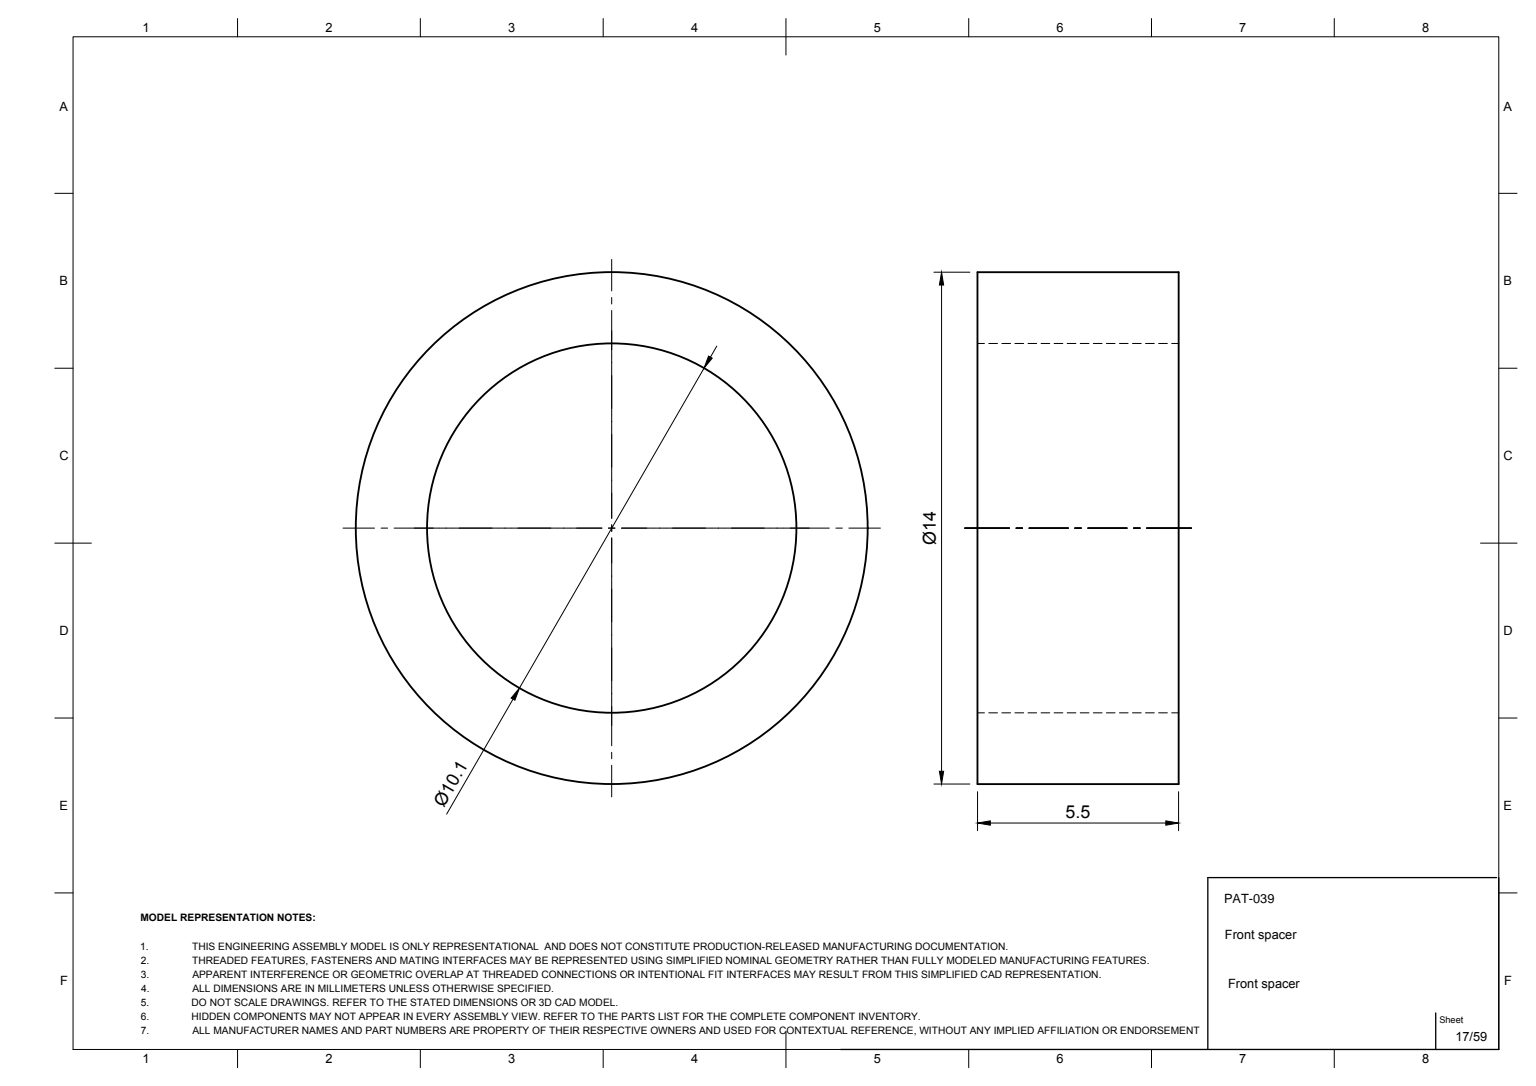
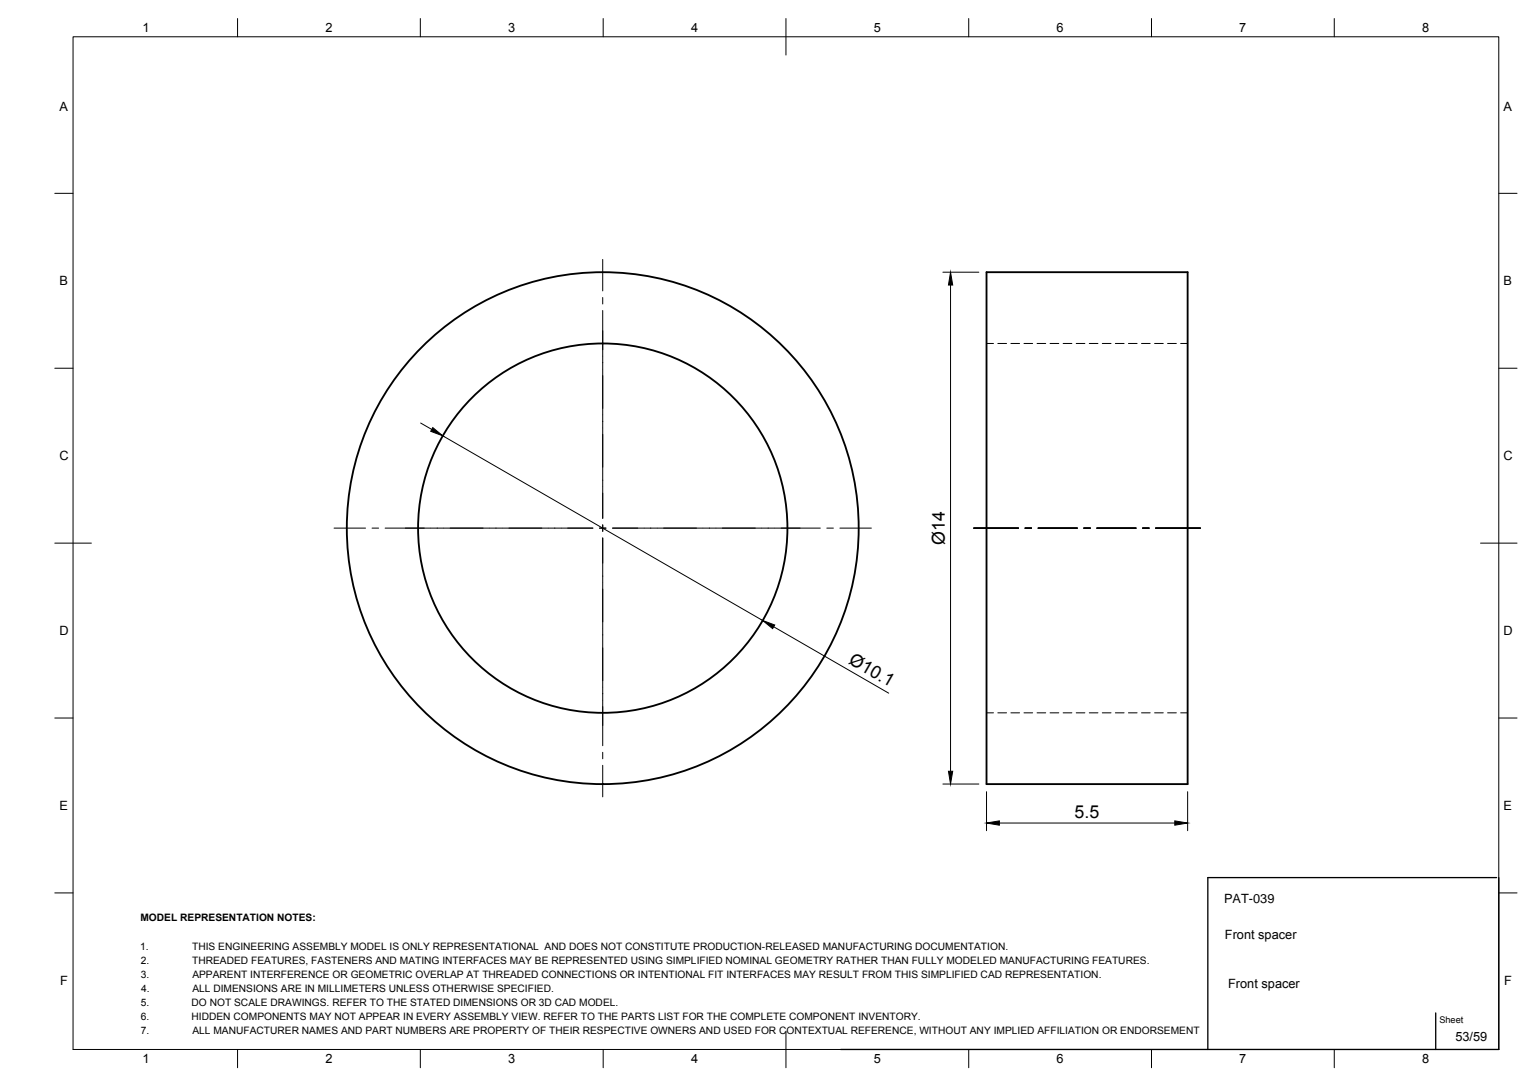
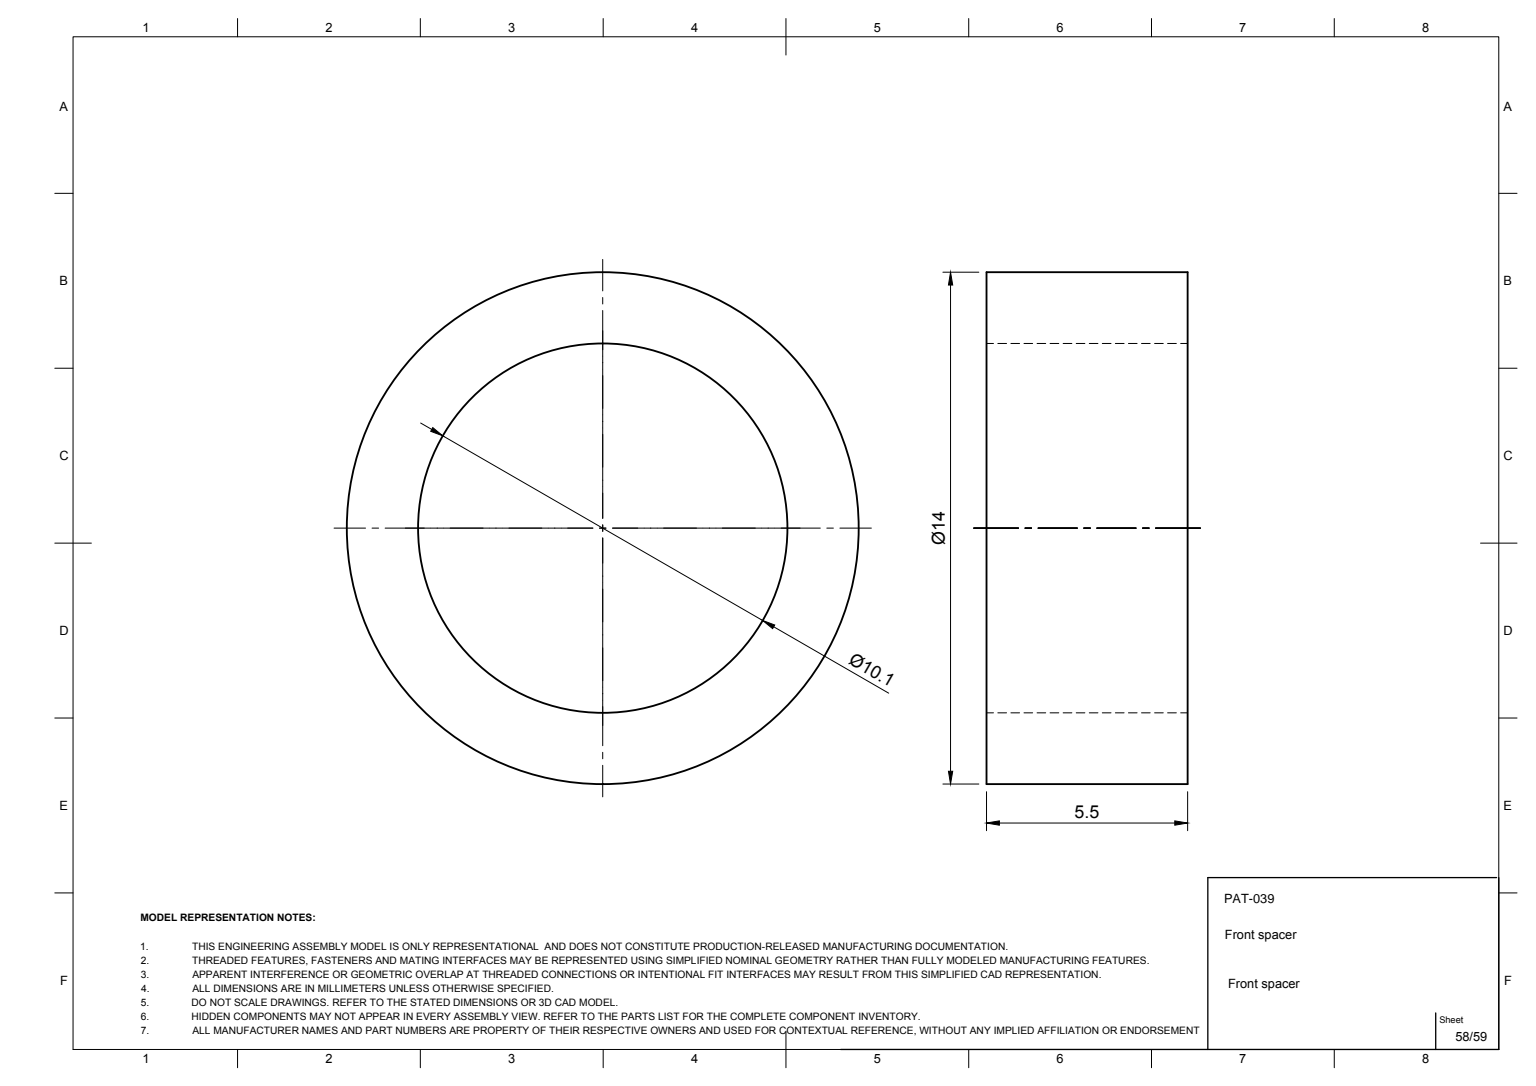
ISO-10303-21;
HEADER;
/* Generated by software containing ST-Developer
 * from STEP Tools, Inc. (www.steptools.com) 
 */

FILE_DESCRIPTION(
/* description */ ('Four-bar parallelogram arm'),
/* implementation_level */ '2;1');

FILE_NAME(
/* name */ 'Front spacer.step',
/* time_stamp */ '2026-10-28T03:24:55-07:00',
/* author */ (''),
/* organization */ (''),
/* preprocessor_version */ 'ST-DEVELOPER v20.2',
/* originating_system */ 'Autodesk Translation Framework v15.17.0.0',
/* authorisation */ '');

FILE_SCHEMA (('AUTOMOTIVE_DESIGN { 1 0 10303 214 3 1 1 }'));
ENDSEC;

DATA;
#10=MECHANICAL_DESIGN_GEOMETRIC_PRESENTATION_REPRESENTATION('',(#634),#14512);
#534=SHAPE_REPRESENTATION_RELATIONSHIP('SRR','None',#14755,#584);
#584=ADVANCED_BREP_SHAPE_REPRESENTATION('',(#692),#14470);
#634=STYLED_ITEM('',(#15080),#692);
#692=MANIFOLD_SOLID_BREP('Body1',#7338);
#798=FACE_BOUND('',#1781,.T.);
#799=FACE_BOUND('',#1783,.T.);
#1057=PLANE('',#8139);
#1058=PLANE('',#8140);
#1295=FACE_OUTER_BOUND('',#1778,.T.);
#1296=FACE_OUTER_BOUND('',#1779,.T.);
#1297=FACE_OUTER_BOUND('',#1780,.T.);
#1298=FACE_OUTER_BOUND('',#1782,.T.);
#1778=EDGE_LOOP('',(#5366,#5367,#5368,#5369));
#1779=EDGE_LOOP('',(#5370,#5371,#5372,#5373));
#1780=EDGE_LOOP('',(#5374));
#1781=EDGE_LOOP('',(#5375));
#1782=EDGE_LOOP('',(#5376));
#1783=EDGE_LOOP('',(#5377));
#2415=LINE('',#11856,#2809);
#2416=LINE('',#11862,#2810);
#2809=VECTOR('',#9467,0.505);
#2810=VECTOR('',#9474,0.7);
#3186=CIRCLE('',#8134,0.505);
#3187=CIRCLE('',#8135,0.505);
#3188=CIRCLE('',#8137,0.7);
#3189=CIRCLE('',#8138,0.7);
#3671=VERTEX_POINT('',#11853);
#3672=VERTEX_POINT('',#11855);
#3673=VERTEX_POINT('',#11859);
#3674=VERTEX_POINT('',#11861);
#4314=EDGE_CURVE('',#3671,#3671,#3186,.T.);
#4315=EDGE_CURVE('',#3671,#3672,#2415,.T.);
#4316=EDGE_CURVE('',#3672,#3672,#3187,.T.);
#4317=EDGE_CURVE('',#3673,#3673,#3188,.T.);
#4318=EDGE_CURVE('',#3673,#3674,#2416,.T.);
#4319=EDGE_CURVE('',#3674,#3674,#3189,.T.);
#5366=ORIENTED_EDGE('',*,*,#4314,.F.);
#5367=ORIENTED_EDGE('',*,*,#4315,.T.);
#5368=ORIENTED_EDGE('',*,*,#4316,.T.);
#5369=ORIENTED_EDGE('',*,*,#4315,.F.);
#5370=ORIENTED_EDGE('',*,*,#4317,.F.);
#5371=ORIENTED_EDGE('',*,*,#4318,.T.);
#5372=ORIENTED_EDGE('',*,*,#4319,.T.);
#5373=ORIENTED_EDGE('',*,*,#4318,.F.);
#5374=ORIENTED_EDGE('',*,*,#4317,.T.);
#5375=ORIENTED_EDGE('',*,*,#4314,.T.);
#5376=ORIENTED_EDGE('',*,*,#4319,.F.);
#5377=ORIENTED_EDGE('',*,*,#4316,.F.);
#6757=CYLINDRICAL_SURFACE('',#8133,0.505);
#6758=CYLINDRICAL_SURFACE('',#8136,0.7);
#7000=ADVANCED_FACE('',(#1295),#6757,.F.);
#7001=ADVANCED_FACE('',(#1296),#6758,.T.);
#7002=ADVANCED_FACE('',(#1297,#798),#1057,.T.);
#7003=ADVANCED_FACE('',(#1298,#799),#1058,.F.);
#7338=CLOSED_SHELL('',(#7000,#7001,#7002,#7003));
#8132=AXIS2_PLACEMENT_3D('',#11851,#9461,#9462);
#8133=AXIS2_PLACEMENT_3D('',#11852,#9463,#9464);
#8134=AXIS2_PLACEMENT_3D('',#11854,#9465,#9466);
#8135=AXIS2_PLACEMENT_3D('',#11857,#9468,#9469);
#8136=AXIS2_PLACEMENT_3D('',#11858,#9470,#9471);
#8137=AXIS2_PLACEMENT_3D('',#11860,#9472,#9473);
#8138=AXIS2_PLACEMENT_3D('',#11863,#9475,#9476);
#8139=AXIS2_PLACEMENT_3D('',#11864,#9477,#9478);
#8140=AXIS2_PLACEMENT_3D('',#11865,#9479,#9480);
#9461=DIRECTION('axis',(0.,0.,1.));
#9462=DIRECTION('refdir',(1.,0.,0.));
#9463=DIRECTION('center_axis',(0.,1.,0.));
#9464=DIRECTION('ref_axis',(1.,0.,0.));
#9465=DIRECTION('center_axis',(0.,-1.,0.));
#9466=DIRECTION('ref_axis',(1.,0.,0.));
#9467=DIRECTION('',(0.,-1.,0.));
#9468=DIRECTION('center_axis',(0.,-1.,0.));
#9469=DIRECTION('ref_axis',(1.,0.,0.));
#9470=DIRECTION('center_axis',(0.,1.,0.));
#9471=DIRECTION('ref_axis',(1.,0.,0.));
#9472=DIRECTION('center_axis',(0.,1.,0.));
#9473=DIRECTION('ref_axis',(1.,0.,0.));
#9474=DIRECTION('',(0.,-1.,0.));
#9475=DIRECTION('center_axis',(0.,1.,0.));
#9476=DIRECTION('ref_axis',(1.,0.,0.));
#9477=DIRECTION('center_axis',(0.,1.,0.));
#9478=DIRECTION('ref_axis',(1.,0.,0.));
#9479=DIRECTION('center_axis',(0.,1.,0.));
#9480=DIRECTION('ref_axis',(1.,0.,0.));
#11851=CARTESIAN_POINT('',(0.,0.,0.));
#11852=CARTESIAN_POINT('Origin',(0.,-1.6,14.));
#11853=CARTESIAN_POINT('',(-0.505,-1.05,14.));
#11854=CARTESIAN_POINT('Origin',(0.,-1.05,14.));
#11855=CARTESIAN_POINT('',(-0.505,-1.6,14.));
#11856=CARTESIAN_POINT('',(-0.505,-1.6,14.));
#11857=CARTESIAN_POINT('Origin',(0.,-1.6,14.));
#11858=CARTESIAN_POINT('Origin',(0.,-1.6,14.));
#11859=CARTESIAN_POINT('',(-0.7,-1.05,14.));
#11860=CARTESIAN_POINT('Origin',(0.,-1.05,14.));
#11861=CARTESIAN_POINT('',(-0.7,-1.6,14.));
#11862=CARTESIAN_POINT('',(-0.7,-1.6,14.));
#11863=CARTESIAN_POINT('Origin',(0.,-1.6,14.));
#11864=CARTESIAN_POINT('Origin',(0.,-1.05,14.));
#11865=CARTESIAN_POINT('Origin',(0.,-1.6,14.));
#14413=UNCERTAINTY_MEASURE_WITH_UNIT(LENGTH_MEASURE(0.001),#14513,
'DISTANCE_ACCURACY_VALUE',
'Maximum model space distance between geometric entities at asserted c
onnectivities');
#14455=UNCERTAINTY_MEASURE_WITH_UNIT(LENGTH_MEASURE(0.001),#14513,
'DISTANCE_ACCURACY_VALUE',
'Maximum model space distance between geometric entities at asserted c
onnectivities');
#14470=(
GEOMETRIC_REPRESENTATION_CONTEXT(3)
GLOBAL_UNCERTAINTY_ASSIGNED_CONTEXT((#14413))
GLOBAL_UNIT_ASSIGNED_CONTEXT((#14513,#14515,#14516))
REPRESENTATION_CONTEXT('','3D')
);
#14512=(
GEOMETRIC_REPRESENTATION_CONTEXT(3)
GLOBAL_UNCERTAINTY_ASSIGNED_CONTEXT((#14455))
GLOBAL_UNIT_ASSIGNED_CONTEXT((#14513,#14515,#14516))
REPRESENTATION_CONTEXT('','3D')
);
#14513=(
LENGTH_UNIT()
NAMED_UNIT(*)
SI_UNIT(.CENTI.,.METRE.)
);
#14515=(
NAMED_UNIT(*)
PLANE_ANGLE_UNIT()
SI_UNIT($,.RADIAN.)
);
#14516=(
NAMED_UNIT(*)
SI_UNIT($,.STERADIAN.)
SOLID_ANGLE_UNIT()
);
#14531=SHAPE_DEFINITION_REPRESENTATION(#14587,#14755);
#14587=PRODUCT_DEFINITION_SHAPE('',$,#14812);
#14755=SHAPE_REPRESENTATION('',(#8132),#14470);
#14797=PRODUCT_DEFINITION_CONTEXT('part definition',#14967,'design');
#14812=PRODUCT_DEFINITION('Front spacer','Front spacer',#14868,#14797);
#14868=PRODUCT_DEFINITION_FORMATION('',$,#14983);
#14967=APPLICATION_CONTEXT(
'Core Data for Automotive Mechanical Design Process');
#14968=PRODUCT_CONTEXT('part definition',#14967,'mechanical');
#14983=PRODUCT('Front spacer','Front spacer','Front spacer',(#14968));
#15074=COLOUR_RGB('Sky Blue',0.24,0.69,0.87);
#15075=FILL_AREA_STYLE_COLOUR('',#15074);
#15076=FILL_AREA_STYLE('',(#15075));
#15077=SURFACE_STYLE_FILL_AREA(#15076);
#15078=SURFACE_SIDE_STYLE('',(#15077));
#15079=SURFACE_STYLE_USAGE(.BOTH.,#15078);
#15080=PRESENTATION_STYLE_ASSIGNMENT((#15079));
ENDSEC;
END-ISO-10303-21;
